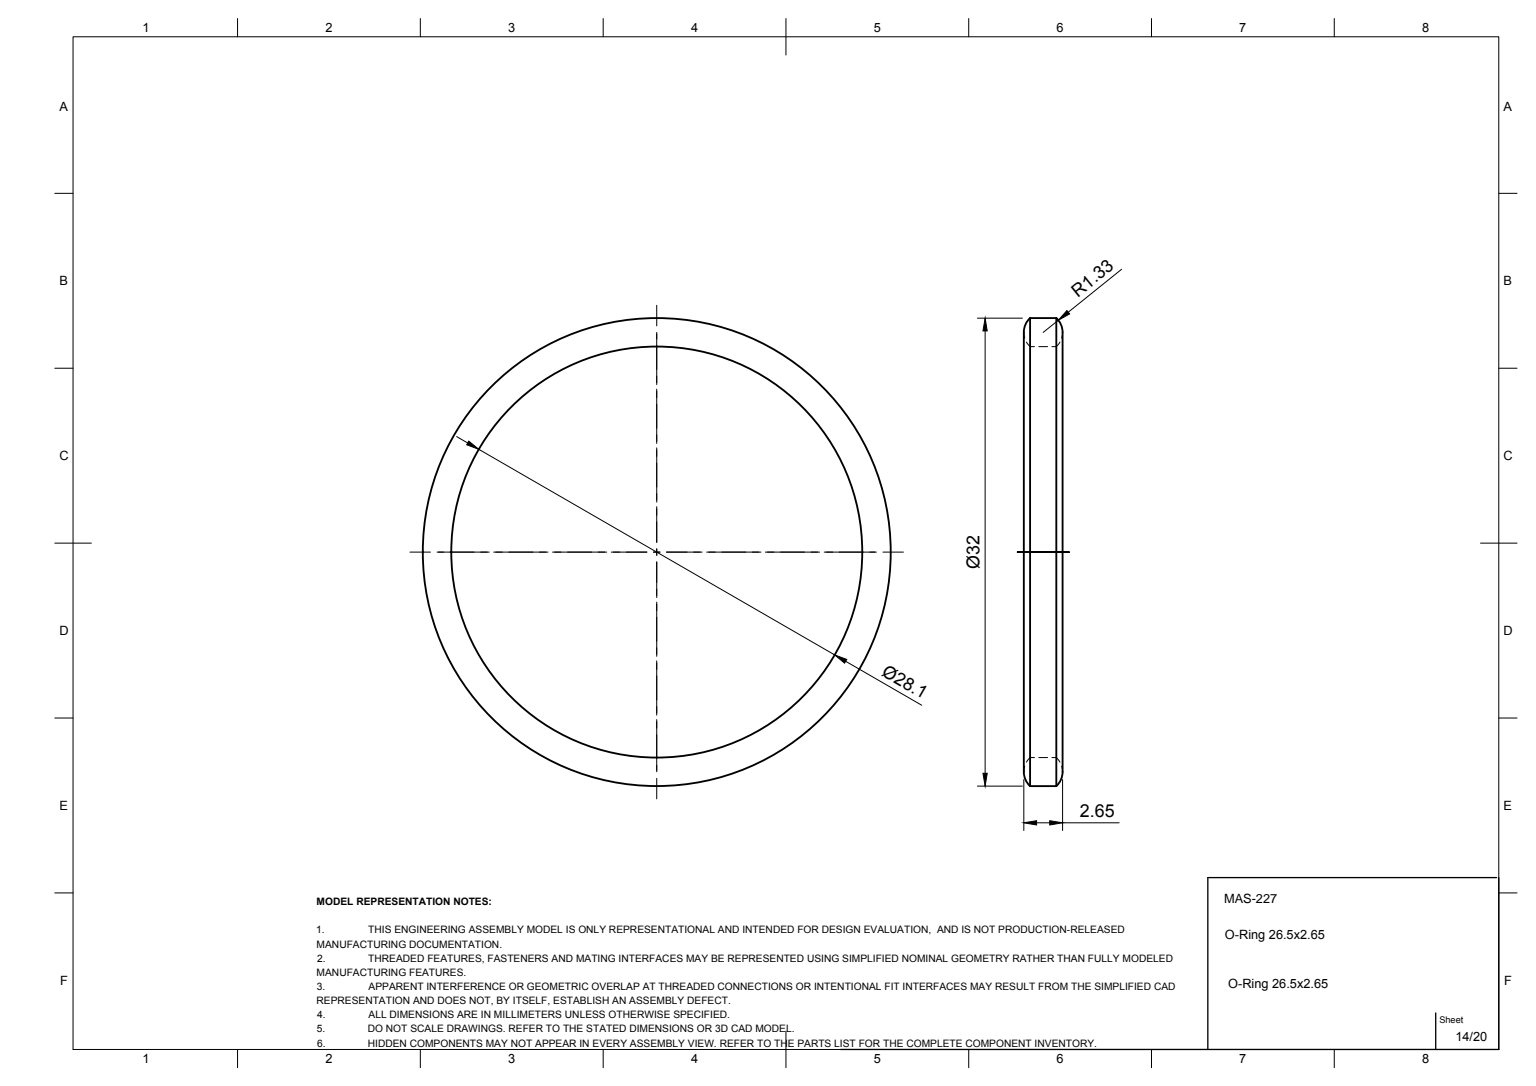
ISO-10303-21;
HEADER;
FILE_DESCRIPTION (('STEP AP214'),
    '1' );
FILE_NAME ( 'O-Ring 26.5x2.65.step', '2026-10-06T08:24:41', ( '' ), ( '' ), 'STEP AP214', 'Unspecified', '' );
FILE_SCHEMA (( 'AUTOMOTIVE_DESIGN' ));
ENDSEC;
DATA;
#16=VECTOR ( 'NONE', #25665, 39.37007874015748143 ) ;
#18=FACE_OUTER_BOUND ( 'NONE', #11254, .T. ) ;
#51=VERTEX_POINT ( 'NONE', #494 ) ;
#141=TOROIDAL_SURFACE ( 'NONE', #14548, 0.5915354330708662012, 0.05216535433070866590 ) ;
#282=DIRECTION ( 'NONE',  ( -5.737213000000000442E-16, 1.000000000000000000, -1.224646799147353207E-16 ) ) ;
#369=CARTESIAN_POINT ( 'NONE',  ( -0.03532354024591771724, -0.6299212598425195653, 0.6299212598425196763 ) ) ;
#494=CARTESIAN_POINT ( 'NONE',  ( -0.03532354024591775193, -0.07677165354330710290, 0.000000000000000000 ) ) ;
#622=CLOSED_SHELL ( 'NONE', ( #8560, #18644, #16249, #1256, #26576, #22771, #9012, #3173 ) ) ;
#701=EDGE_CURVE ( 'NONE', #51, #18891, #12838, .T. ) ;
#703=CARTESIAN_POINT ( 'NONE',  ( 0.03532354024591842501, -0.6299212598425196763, 0.000000000000000000 ) ) ;
#723=EDGE_CURVE ( 'NONE', #11887, #24760, #20053, .T. ) ;
#745=LINE ( 'NONE', #11474, #16 ) ;
#917=CARTESIAN_POINT ( 'NONE',  ( 3.387491338582676985E-16, -0.6299212598425196763, 0.000000000000000000 ) ) ;
#1221=PRODUCT_DEFINITION_SHAPE ( 'NONE', 'NONE',  #2566 ) ;
#1256=ADVANCED_FACE ( 'NONE', ( #5909 ), #16077, .T. ) ;
#1277=DIRECTION ( 'NONE',  ( 1.000000000000000000, 0.000000000000000000, 0.000000000000000000 ) ) ;
#1308=ORIENTED_EDGE ( 'NONE', *, *, #23601, .T. ) ;
#1320=EDGE_CURVE ( 'NONE', #51, #1745, #8572, .T. ) ;
#1375=DIRECTION ( 'NONE',  ( 5.737213000000000442E-16, -1.000000000000000000, 0.000000000000000000 ) ) ;
#1377=EDGE_CURVE ( 'NONE', #25529, #10943, #6997, .T. ) ;
#1378=DIRECTION ( 'NONE',  ( 1.000000000000000000, 0.000000000000000000, 0.000000000000000000 ) ) ;
#1561=CARTESIAN_POINT ( 'NONE',  ( 0.03532354024591839031, -0.6299212598425196763, -0.5531496062992127261 ) ) ;
#1621=ORIENTED_EDGE ( 'NONE', *, *, #19395, .F. ) ;
#1686=DIRECTION ( 'NONE',  ( -5.737213000000000442E-16, 1.000000000000000000, -1.224646799147353207E-16 ) ) ;
#1727=LINE ( 'NONE', #7814, #20994 ) ;
#1729=ORIENTED_EDGE ( 'NONE', *, *, #3922, .F. ) ;
#1745=VERTEX_POINT ( 'NONE', #5410 ) ;
#1841=CIRCLE ( 'NONE', #24842, 0.5531496062992126150 ) ;
#1899=SURFACE_SIDE_STYLE ('',( #20830 ) ) ;
#1912=DIRECTION ( 'NONE',  ( 1.000000000000000000, 0.000000000000000000, 0.000000000000000000 ) ) ;
#2140=DIRECTION ( 'NONE',  ( 0.000000000000000000, 1.000000000000000000, 0.000000000000000000 ) ) ;
#2162=AXIS2_PLACEMENT_3D ( 'NONE', #917, #9504, #7127 ) ;
#2367=CIRCLE ( 'NONE', #19974, 0.6299212598425196763 ) ;
#2507=CARTESIAN_POINT ( 'NONE',  ( 0.03532354024591842501, 0.000000000000000000, 0.000000000000000000 ) ) ;
#2559=EDGE_CURVE ( 'NONE', #27334, #51, #15612, .T. ) ;
#2561=CARTESIAN_POINT ( 'NONE',  ( 3.387491338582676985E-16, -0.6299212598425196763, 0.000000000000000000 ) ) ;
#2566=PRODUCT_DEFINITION ( 'UNKNOWN', '', #22916, #5726 ) ;
#2676=DIRECTION ( 'NONE',  ( 0.000000000000000000, 1.000000000000000000, 0.000000000000000000 ) ) ;
#3100=CYLINDRICAL_SURFACE ( 'NONE', #26407, 0.6299212598425196763 ) ;
#3173=ADVANCED_FACE ( 'NONE', ( #17968 ), #22023, .T. ) ;
#3194=DIRECTION ( 'NONE',  ( 0.000000000000000000, 1.000000000000000000, 0.000000000000000000 ) ) ;
#3206=DIRECTION ( 'NONE',  ( 0.000000000000000000, 1.000000000000000000, 0.000000000000000000 ) ) ;
#3358=DIRECTION ( 'NONE',  ( 0.000000000000000000, 1.000000000000000000, 0.000000000000000000 ) ) ;
#3457=DIRECTION ( 'NONE',  ( 5.737213000000000442E-16, -1.000000000000000000, 0.000000000000000000 ) ) ;
#3491=CYLINDRICAL_SURFACE ( 'NONE', #18443, 0.5531496062992126150 ) ;
#3649=APPLICATION_CONTEXT ( 'automotive_design' ) ;
#3665=DIRECTION ( 'NONE',  ( 0.000000000000000000, 0.000000000000000000, 1.000000000000000000 ) ) ;
#3722=CIRCLE ( 'NONE', #22210, 0.6299212598425196763 ) ;
#3837=CIRCLE ( 'NONE', #25481, 0.6299212598425196763 ) ;
#3861=EDGE_CURVE ( 'NONE', #26623, #1745, #13934, .T. ) ;
#3922=EDGE_CURVE ( 'NONE', #11887, #24839, #745, .T. ) ;
#3923=CIRCLE ( 'NONE', #15647, 0.5531496062992126150 ) ;
#3950=DIRECTION ( 'NONE',  ( 1.000000000000000000, 0.000000000000000000, 0.000000000000000000 ) ) ;
#3983=ORIENTED_EDGE ( 'NONE', *, *, #3922, .T. ) ;
#4113=ORIENTED_EDGE ( 'NONE', *, *, #7145, .F. ) ;
#4133=ORIENTED_EDGE ( 'NONE', *, *, #2559, .T. ) ;
#4199=CARTESIAN_POINT ( 'NONE',  ( 0.03532354024591839031, -0.6299212598425196763, 0.000000000000000000 ) ) ;
#4249=CIRCLE ( 'NONE', #25904, 0.05216535433070866590 ) ;
#4542=DIRECTION ( 'NONE',  ( 1.000000000000000000, 0.000000000000000000, 0.000000000000000000 ) ) ;
#4793=DIRECTION ( 'NONE',  ( 1.000000000000000000, 0.000000000000000000, 0.000000000000000000 ) ) ;
#4849=ORIENTED_EDGE ( 'NONE', *, *, #1377, .T. ) ;
#5188=ORIENTED_EDGE ( 'NONE', *, *, #10508, .T. ) ;
#5229=CARTESIAN_POINT ( 'NONE',  ( 0.000000000000000000, 0.000000000000000000, 0.000000000000000000 ) ) ;
#5323=CARTESIAN_POINT ( 'NONE',  ( 0.03532354024591842501, -0.6299212598425196763, 0.000000000000000000 ) ) ;
#5348=ORIENTED_EDGE ( 'NONE', *, *, #9549, .T. ) ;
#5410=CARTESIAN_POINT ( 'NONE',  ( 0.03532354024591839031, -0.07677165354330710290, 0.000000000000000000 ) ) ;
#5496=ORIENTED_EDGE ( 'NONE', *, *, #25810, .T. ) ;
#5510=PRODUCT ( 'O-Ring 26.5x2.65', 'O-Ring 26.5x2.65', '', ( #21672 ) ) ;
#5527=EDGE_CURVE ( 'NONE', #24760, #25529, #17543, .T. ) ;
#5576=AXIS2_PLACEMENT_3D ( 'NONE', #16947, #3950, #3358 ) ;
#5726=PRODUCT_DEFINITION_CONTEXT ( 'detailed design', #25319, 'design' ) ;
#5782=CARTESIAN_POINT ( 'NONE',  ( 3.168943700787402105E-16, -0.6299212598425196763, 0.000000000000000000 ) ) ;
#5828=CIRCLE ( 'NONE', #11673, 0.5531496062992126150 ) ;
#5871=ORIENTED_EDGE ( 'NONE', *, *, #7145, .T. ) ;
#5874=PRESENTATION_STYLE_ASSIGNMENT (( #23395 ) ) ;
#5909=FACE_OUTER_BOUND ( 'NONE', #24647, .T. ) ;
#5934=CARTESIAN_POINT ( 'NONE',  ( 0.03532354024591842501, -1.259842519685039353, 7.714310545810098438E-17 ) ) ;
#5938=LINE ( 'NONE', #7912, #15070 ) ;
#6195=DIMENSIONAL_EXPONENTS ( 1.000000000000000000, 0.000000000000000000, 0.000000000000000000, 0.000000000000000000, 0.000000000000000000, 0.000000000000000000, 0.000000000000000000 ) ;
#6290=( LENGTH_UNIT ( ) NAMED_UNIT ( * ) SI_UNIT ( $, .METRE. ) ) ;
#6293=ORIENTED_EDGE ( 'NONE', *, *, #24317, .F. ) ;
#6388=STYLED_ITEM ( 'NONE', ( #5874 ), #12535 ) ;
#6407=ORIENTED_EDGE ( 'NONE', *, *, #24317, .T. ) ;
#6613=ORIENTED_EDGE ( 'NONE', *, *, #9048, .F. ) ;
#6845=MECHANICAL_DESIGN_GEOMETRIC_PRESENTATION_REPRESENTATION('',(#6388),#8635);
#6878=ORIENTED_EDGE ( 'NONE', *, *, #1320, .T. ) ;
#6892=ORIENTED_EDGE ( 'NONE', *, *, #24202, .T. ) ;
#6938=CARTESIAN_POINT ( 'NONE',  ( 0.03532354024591839031, -1.183070866141732402, 6.774128948039492984E-17 ) ) ;
#6978=AXIS2_PLACEMENT_3D ( 'NONE', #20907, #22894, #25283 ) ;
#6997=CIRCLE ( 'NONE', #24127, 0.6299212598425196763 ) ;
#7054=CARTESIAN_POINT ( 'NONE',  ( -0.03532354024591775193, -1.183070866141732402, 6.774128948039492984E-17 ) ) ;
#7127=DIRECTION ( 'NONE',  ( 0.000000000000000000, 0.000000000000000000, -1.000000000000000000 ) ) ;
#7145=EDGE_CURVE ( 'NONE', #18891, #19141, #26171, .T. ) ;
#7197=FACE_OUTER_BOUND ( 'NONE', #21819, .T. ) ;
#7289=DIRECTION ( 'NONE',  ( 0.000000000000000000, 1.000000000000000000, 0.000000000000000000 ) ) ;
#7307=AXIS2_PLACEMENT_3D ( 'NONE', #9577, #20051, #20188 ) ;
#7358=CARTESIAN_POINT ( 'NONE',  ( 3.606039370078740678E-16, -0.6299212598425196763, 0.000000000000000000 ) ) ;
#7437=DIRECTION ( 'NONE',  ( 1.000000000000000000, 0.000000000000000000, 0.000000000000000000 ) ) ;
#7561=ORIENTED_EDGE ( 'NONE', *, *, #20852, .T. ) ;
#7745=DIRECTION ( 'NONE',  ( 0.000000000000000000, 1.000000000000000000, 0.000000000000000000 ) ) ;
#7814=CARTESIAN_POINT ( 'NONE',  ( 3.606039370078740678E-16, 0.000000000000000000, 0.000000000000000000 ) ) ;
#7894=DIRECTION ( 'NONE',  ( 1.000000000000000000, 0.000000000000000000, 0.000000000000000000 ) ) ;
#7912=CARTESIAN_POINT ( 'NONE',  ( 3.168943700787402105E-16, -1.183070866141732402, 6.774128948039492984E-17 ) ) ;
#7923=DIRECTION ( 'NONE',  ( 1.000000000000000000, 0.000000000000000000, 0.000000000000000000 ) ) ;
#8115=CARTESIAN_POINT ( 'NONE',  ( -0.03532354024591771724, -0.6299212598425196763, 0.000000000000000000 ) ) ;
#8193=DIRECTION ( 'NONE',  ( -1.000000000000000000, 0.000000000000000000, 0.000000000000000000 ) ) ;
#8226=CARTESIAN_POINT ( 'NONE',  ( -0.03532354024591775193, -0.6299212598425196763, 0.000000000000000000 ) ) ;
#8367=AXIS2_PLACEMENT_3D ( 'NONE', #19784, #4793, #2676 ) ;
#8370=DIRECTION ( 'NONE',  ( 0.000000000000000000, 1.000000000000000000, 0.000000000000000000 ) ) ;
#8452=ORIENTED_EDGE ( 'NONE', *, *, #15845, .T. ) ;
#8560=ADVANCED_FACE ( 'NONE', ( #10919 ), #141, .T. ) ;
#8572=LINE ( 'NONE', #21570, #16465 ) ;
#8584=( LENGTH_UNIT ( ) NAMED_UNIT ( * ) SI_UNIT ( $, .METRE. ) ) ;
#8595=CARTESIAN_POINT ( 'NONE',  ( -0.03532354024591775193, -0.6299212598425196763, 0.000000000000000000 ) ) ;
#8635=( GEOMETRIC_REPRESENTATION_CONTEXT ( 3 ) GLOBAL_UNCERTAINTY_ASSIGNED_CONTEXT ( ( #20622 ) ) GLOBAL_UNIT_ASSIGNED_CONTEXT ( ( #10223, #14502, #18839 ) ) REPRESENTATION_CONTEXT ( 'NONE', 'WORKASPACE' ) ) ;
#8706=ORIENTED_EDGE ( 'NONE', *, *, #3861, .T. ) ;
#8817=ORIENTED_EDGE ( 'NONE', *, *, #3861, .F. ) ;
#8923=DIRECTION ( 'NONE',  ( 1.000000000000000000, 5.737213000000000442E-16, 0.000000000000000000 ) ) ;
#8965=AXIS2_PLACEMENT_3D ( 'NONE', #10400, #14533, #19018 ) ;
#9012=ADVANCED_FACE ( 'NONE', ( #7197 ), #18185, .F. ) ;
#9048=EDGE_CURVE ( 'NONE', #19937, #24839, #3722, .T. ) ;
#9159=TOROIDAL_SURFACE ( 'NONE', #15501, 0.5915354330708662012, 0.05216535433070866590 ) ;
#9460=TOROIDAL_SURFACE ( 'NONE', #18012, 0.5915354330708662012, 0.05216535433070866590 ) ;
#9504=DIRECTION ( 'NONE',  ( 1.000000000000000000, 5.737213000000000442E-16, 0.000000000000000000 ) ) ;
#9549=EDGE_CURVE ( 'NONE', #10943, #11887, #2367, .T. ) ;
#9577=CARTESIAN_POINT ( 'NONE',  ( 3.168943700787402105E-16, -0.6299212598425196763, 0.000000000000000000 ) ) ;
#9708=CARTESIAN_POINT ( 'NONE',  ( -0.03532354024591771724, -0.6299212598425196763, 0.000000000000000000 ) ) ;
#10152=CARTESIAN_POINT ( 'NONE',  ( 3.387491338582676492E-16, -0.6299212598425195653, 0.5915354330708662012 ) ) ;
#10223=( CONVERSION_BASED_UNIT ( 'INCH', #18990 ) LENGTH_UNIT ( ) NAMED_UNIT ( #6195 ) ) ;
#10261=DIRECTION ( 'NONE',  ( 1.000000000000000000, 0.000000000000000000, 0.000000000000000000 ) ) ;
#10400=CARTESIAN_POINT ( 'NONE',  ( 0.03532354024591839031, -0.6299212598425196763, 0.000000000000000000 ) ) ;
#10445=COLOUR_RGB ( '', 0.31764706, 0.68627451, 0.89019608) ;
#10475=AXIS2_PLACEMENT_3D ( 'NONE', #19178, #282, #16785 ) ;
#10508=EDGE_CURVE ( 'NONE', #18891, #10943, #22660, .T. ) ;
#10552=( NAMED_UNIT ( * ) PLANE_ANGLE_UNIT ( ) SI_UNIT ( $, .RADIAN. ) ) ;
#10610=DIRECTION ( 'NONE',  ( 1.000000000000000000, 0.000000000000000000, 0.000000000000000000 ) ) ;
#10700=( NAMED_UNIT ( * ) SI_UNIT ( $, .STERADIAN. ) SOLID_ANGLE_UNIT ( ) ) ;
#10913=ORIENTED_EDGE ( 'NONE', *, *, #701, .T. ) ;
#10919=FACE_OUTER_BOUND ( 'NONE', #21859, .T. ) ;
#10943=VERTEX_POINT ( 'NONE', #369 ) ;
#11074=CIRCLE ( 'NONE', #8367, 0.6299212598425196763 ) ;
#11125=DIRECTION ( 'NONE',  ( 0.000000000000000000, 1.000000000000000000, 0.000000000000000000 ) ) ;
#11254=EDGE_LOOP ( 'NONE', ( #27328, #5871, #12556, #15233, #16781, #13315 ) ) ;
#11343=ORIENTED_EDGE ( 'NONE', *, *, #1377, .F. ) ;
#11417=ORIENTED_EDGE ( 'NONE', *, *, #25810, .F. ) ;
#11474=CARTESIAN_POINT ( 'NONE',  ( 3.606039370078740678E-16, -1.259842519685039353, 7.714310545810098438E-17 ) ) ;
#11588=AXIS2_PLACEMENT_3D ( 'NONE', #5229, #3665, #7923 ) ;
#11673=AXIS2_PLACEMENT_3D ( 'NONE', #27494, #1912, #14660 ) ;
#11887=VERTEX_POINT ( 'NONE', #20844 ) ;
#12159=EDGE_CURVE ( 'NONE', #22507, #26151, #1841, .T. ) ;
#12245=ORIENTED_EDGE ( 'NONE', *, *, #701, .F. ) ;
#12535=MANIFOLD_SOLID_BREP ( 'O-Ring 26.5x2.65', #622 ) ;
#12556=ORIENTED_EDGE ( 'NONE', *, *, #18908, .T. ) ;
#12838=CIRCLE ( 'NONE', #6978, 0.5531496062992126150 ) ;
#13036=DIRECTION ( 'NONE',  ( 1.000000000000000000, 5.737213000000000442E-16, 0.000000000000000000 ) ) ;
#13038=ORIENTED_EDGE ( 'NONE', *, *, #20852, .F. ) ;
#13084=ORIENTED_EDGE ( 'NONE', *, *, #25064, .T. ) ;
#13315=ORIENTED_EDGE ( 'NONE', *, *, #9549, .F. ) ;
#13403=DIMENSIONAL_EXPONENTS ( 1.000000000000000000, 0.000000000000000000, 0.000000000000000000, 0.000000000000000000, 0.000000000000000000, 0.000000000000000000, 0.000000000000000000 ) ;
#13446=EDGE_CURVE ( 'NONE', #19463, #18018, #19077, .T. ) ;
#13454=AXIS2_PLACEMENT_3D ( 'NONE', #9708, #20867, #3194 ) ;
#13637=ORIENTED_EDGE ( 'NONE', *, *, #12159, .F. ) ;
#13748=ORIENTED_EDGE ( 'NONE', *, *, #2559, .F. ) ;
#13856=DIRECTION ( 'NONE',  ( 0.000000000000000000, 1.000000000000000000, 0.000000000000000000 ) ) ;
#13932=CARTESIAN_POINT ( 'NONE',  ( -0.03532354024591775193, -0.6299212598425196763, 0.000000000000000000 ) ) ;
#13934=CIRCLE ( 'NONE', #8965, 0.5531496062992126150 ) ;
#14012=EDGE_CURVE ( 'NONE', #19141, #26151, #5938, .T. ) ;
#14091=DIRECTION ( 'NONE',  ( 1.000000000000000000, 0.000000000000000000, 0.000000000000000000 ) ) ;
#14222=AXIS2_PLACEMENT_3D ( 'NONE', #16221, #1378, #7745 ) ;
#14424=DIRECTION ( 'NONE',  ( 1.000000000000000000, 0.000000000000000000, 0.000000000000000000 ) ) ;
#14502=( NAMED_UNIT ( * ) PLANE_ANGLE_UNIT ( ) SI_UNIT ( $, .RADIAN. ) ) ;
#14533=DIRECTION ( 'NONE',  ( 1.000000000000000000, 0.000000000000000000, 0.000000000000000000 ) ) ;
#14548=AXIS2_PLACEMENT_3D ( 'NONE', #2561, #13036, #19808 ) ;
#14660=DIRECTION ( 'NONE',  ( 0.000000000000000000, 1.000000000000000000, 0.000000000000000000 ) ) ;
#14685=DIRECTION ( 'NONE',  ( 0.000000000000000000, 1.000000000000000000, 0.000000000000000000 ) ) ;
#14716=EDGE_LOOP ( 'NONE', ( #24966, #25552, #7561, #8706, #23121, #13748 ) ) ;
#14734=AXIS2_PLACEMENT_3D ( 'NONE', #8226, #4542, #8370 ) ;
#14830=DIRECTION ( 'NONE',  ( 1.000000000000000000, 5.737213000000000442E-16, 0.000000000000000000 ) ) ;
#15070=VECTOR ( 'NONE', #14424, 39.37007874015748143 ) ;
#15138=ORIENTED_EDGE ( 'NONE', *, *, #13446, .F. ) ;
#15233=ORIENTED_EDGE ( 'NONE', *, *, #19395, .T. ) ;
#15501=AXIS2_PLACEMENT_3D ( 'NONE', #23441, #14830, #25820 ) ;
#15612=CIRCLE ( 'NONE', #14734, 0.5531496062992126150 ) ;
#15647=AXIS2_PLACEMENT_3D ( 'NONE', #13932, #25725, #7289 ) ;
#15747=CARTESIAN_POINT ( 'NONE',  ( -0.03532354024591775193, -0.6299212598425196763, -0.5531496062992126150 ) ) ;
#15817=DIRECTION ( 'NONE',  ( 1.000000000000000000, 0.000000000000000000, 0.000000000000000000 ) ) ;
#15845=EDGE_CURVE ( 'NONE', #25529, #18018, #1727, .T. ) ;
#15977=DIRECTION ( 'NONE',  ( 1.000000000000000000, 0.000000000000000000, 0.000000000000000000 ) ) ;
#16077=CYLINDRICAL_SURFACE ( 'NONE', #14222, 0.6299212598425196763 ) ;
#16221=CARTESIAN_POINT ( 'NONE',  ( 3.606039370078740678E-16, -0.6299212598425196763, 0.000000000000000000 ) ) ;
#16249=ADVANCED_FACE ( 'NONE', ( #21656 ), #9460, .T. ) ;
#16465=VECTOR ( 'NONE', #10261, 39.37007874015748143 ) ;
#16570=( GEOMETRIC_REPRESENTATION_CONTEXT ( 3 ) GLOBAL_UNCERTAINTY_ASSIGNED_CONTEXT ( ( #23243 ) ) GLOBAL_UNIT_ASSIGNED_CONTEXT ( ( #25683, #10552, #10700 ) ) REPRESENTATION_CONTEXT ( 'NONE', 'WORKASPACE' ) ) ;
#16606=DIRECTION ( 'NONE',  ( 1.000000000000000000, 0.000000000000000000, 0.000000000000000000 ) ) ;
#16655=ORIENTED_EDGE ( 'NONE', *, *, #9048, .T. ) ;
#16781=ORIENTED_EDGE ( 'NONE', *, *, #723, .F. ) ;
#16785=DIRECTION ( 'NONE',  ( -1.000000000000000000, 0.000000000000000000, 0.000000000000000000 ) ) ;
#16820=ORIENTED_EDGE ( 'NONE', *, *, #14012, .F. ) ;
#16855=DIRECTION ( 'NONE',  ( 1.000000000000000000, 0.000000000000000000, 0.000000000000000000 ) ) ;
#16933=ORIENTED_EDGE ( 'NONE', *, *, #723, .T. ) ;
#16947=CARTESIAN_POINT ( 'NONE',  ( 0.03532354024591839031, -0.6299212598425196763, 0.000000000000000000 ) ) ;
#17115=EDGE_LOOP ( 'NONE', ( #4133, #10913, #5188, #11343, #21481, #1621 ) ) ;
#17259=CARTESIAN_POINT ( 'NONE',  ( 0.03532354024591842501, -0.6299212598425196763, 0.000000000000000000 ) ) ;
#17353=DIRECTION ( 'NONE',  ( 1.000000000000000000, 0.000000000000000000, 0.000000000000000000 ) ) ;
#17473=ORIENTED_EDGE ( 'NONE', *, *, #12159, .T. ) ;
#17543=CIRCLE ( 'NONE', #13454, 0.6299212598425196763 ) ;
#17968=FACE_OUTER_BOUND ( 'NONE', #26843, .T. ) ;
#17990=CARTESIAN_POINT ( 'NONE',  ( 0.03532354024591842501, -0.6299212598425196763, -0.6299212598425196763 ) ) ;
#18012=AXIS2_PLACEMENT_3D ( 'NONE', #19676, #8923, #26164 ) ;
#18018=VERTEX_POINT ( 'NONE', #2507 ) ;
#18054=FACE_OUTER_BOUND ( 'NONE', #27815, .T. ) ;
#18185=CYLINDRICAL_SURFACE ( 'NONE', #7307, 0.5531496062992126150 ) ;
#18443=AXIS2_PLACEMENT_3D ( 'NONE', #5782, #7894, #3206 ) ;
#18644=ADVANCED_FACE ( 'NONE', ( #26812 ), #3491, .F. ) ;
#18649=CARTESIAN_POINT ( 'NONE',  ( -0.03532354024591771724, 0.000000000000000000, 0.000000000000000000 ) ) ;
#18757=CIRCLE ( 'NONE', #21475, 0.05216535433070866590 ) ;
#18767=ADVANCED_BREP_SHAPE_REPRESENTATION ( 'O-Ring 26.5x2.65', ( #12535, #11588 ), #16570 ) ;
#18839=( NAMED_UNIT ( * ) SI_UNIT ( $, .STERADIAN. ) SOLID_ANGLE_UNIT ( ) ) ;
#18891=VERTEX_POINT ( 'NONE', #26884 ) ;
#18896=ORIENTED_EDGE ( 'NONE', *, *, #5527, .T. ) ;
#18905=ORIENTED_EDGE ( 'NONE', *, *, #13446, .T. ) ;
#18908=EDGE_CURVE ( 'NONE', #19141, #27334, #3923, .T. ) ;
#18960=CARTESIAN_POINT ( 'NONE',  ( 0.03532354024591842501, -0.6299212598425195653, 0.6299212598425196763 ) ) ;
#18990=LENGTH_MEASURE_WITH_UNIT ( LENGTH_MEASURE( 0.02539999999999999897 ), #6290 ) ;
#19018=DIRECTION ( 'NONE',  ( 0.000000000000000000, 1.000000000000000000, 0.000000000000000000 ) ) ;
#19077=CIRCLE ( 'NONE', #22216, 0.6299212598425196763 ) ;
#19141=VERTEX_POINT ( 'NONE', #7054 ) ;
#19176=SHAPE_REPRESENTATION_RELATIONSHIP ( 'NONE' , 'NONE' ,  #27787, #18767 ) ;
#19178=CARTESIAN_POINT ( 'NONE',  ( 3.387491338582676492E-16, -0.6299212598425195653, 0.5915354330708662012 ) ) ;
#19395=EDGE_CURVE ( 'NONE', #27334, #24760, #18757, .T. ) ;
#19463=VERTEX_POINT ( 'NONE', #17990 ) ;
#19676=CARTESIAN_POINT ( 'NONE',  ( 3.387491338582676985E-16, -0.6299212598425196763, 0.000000000000000000 ) ) ;
#19784=CARTESIAN_POINT ( 'NONE',  ( 0.03532354024591842501, -0.6299212598425196763, 0.000000000000000000 ) ) ;
#19808=DIRECTION ( 'NONE',  ( 0.000000000000000000, 0.000000000000000000, -1.000000000000000000 ) ) ;
#19937=VERTEX_POINT ( 'NONE', #18960 ) ;
#19974=AXIS2_PLACEMENT_3D ( 'NONE', #8115, #20819, #23093 ) ;
#20051=DIRECTION ( 'NONE',  ( 1.000000000000000000, 0.000000000000000000, 0.000000000000000000 ) ) ;
#20053=CIRCLE ( 'NONE', #20968, 0.6299212598425196763 ) ;
#20188=DIRECTION ( 'NONE',  ( 0.000000000000000000, 1.000000000000000000, 0.000000000000000000 ) ) ;
#20622=UNCERTAINTY_MEASURE_WITH_UNIT (LENGTH_MEASURE( 1.000000000000000082E-05 ), #10223, 'distance_accuracy_value', 'NONE') ;
#20786=ORIENTED_EDGE ( 'NONE', *, *, #15845, .F. ) ;
#20819=DIRECTION ( 'NONE',  ( 1.000000000000000000, 0.000000000000000000, 0.000000000000000000 ) ) ;
#20830=SURFACE_STYLE_FILL_AREA ( #27763 ) ;
#20844=CARTESIAN_POINT ( 'NONE',  ( -0.03532354024591771724, -1.259842519685039353, 7.714310545810098438E-17 ) ) ;
#20852=EDGE_CURVE ( 'NONE', #26151, #26623, #5828, .T. ) ;
#20867=DIRECTION ( 'NONE',  ( 1.000000000000000000, 0.000000000000000000, 0.000000000000000000 ) ) ;
#20907=CARTESIAN_POINT ( 'NONE',  ( -0.03532354024591775193, -0.6299212598425196763, 0.000000000000000000 ) ) ;
#20968=AXIS2_PLACEMENT_3D ( 'NONE', #25140, #1277, #22604 ) ;
#20994=VECTOR ( 'NONE', #16855, 39.37007874015748143 ) ;
#21019=LENGTH_MEASURE_WITH_UNIT ( LENGTH_MEASURE( 0.02539999999999999897 ), #8584 ) ;
#21475=AXIS2_PLACEMENT_3D ( 'NONE', #24819, #1375, #14091 ) ;
#21481=ORIENTED_EDGE ( 'NONE', *, *, #5527, .F. ) ;
#21570=CARTESIAN_POINT ( 'NONE',  ( 3.168943700787402105E-16, -0.07677165354330710290, 0.000000000000000000 ) ) ;
#21656=FACE_OUTER_BOUND ( 'NONE', #17115, .T. ) ;
#21672=PRODUCT_CONTEXT ( 'NONE', #3649, 'mechanical' ) ;
#21819=EDGE_LOOP ( 'NONE', ( #16820, #4113, #12245, #6878, #1308, #17473 ) ) ;
#21830=CIRCLE ( 'NONE', #24529, 0.05216535433070866590 ) ;
#21859=EDGE_LOOP ( 'NONE', ( #13084, #6892, #27343, #8817, #6293, #18905 ) ) ;
#21889=CARTESIAN_POINT ( 'NONE',  ( 0.03532354024591839031, -0.6299212598425196763, 0.5531496062992127261 ) ) ;
#22023=TOROIDAL_SURFACE ( 'NONE', #2162, 0.5915354330708662012, 0.05216535433070866590 ) ;
#22210=AXIS2_PLACEMENT_3D ( 'NONE', #703, #15817, #26678 ) ;
#22216=AXIS2_PLACEMENT_3D ( 'NONE', #17259, #10610, #2140 ) ;
#22507=VERTEX_POINT ( 'NONE', #21889 ) ;
#22604=DIRECTION ( 'NONE',  ( 0.000000000000000000, 1.000000000000000000, 0.000000000000000000 ) ) ;
#22660=CIRCLE ( 'NONE', #10475, 0.05216535433070866590 ) ;
#22771=ADVANCED_FACE ( 'NONE', ( #18 ), #9159, .T. ) ;
#22894=DIRECTION ( 'NONE',  ( 1.000000000000000000, 0.000000000000000000, 0.000000000000000000 ) ) ;
#22916=PRODUCT_DEFINITION_FORMATION_WITH_SPECIFIED_SOURCE ( 'ANY', '', #5510, .NOT_KNOWN. ) ;
#23093=DIRECTION ( 'NONE',  ( 0.000000000000000000, 1.000000000000000000, 0.000000000000000000 ) ) ;
#23121=ORIENTED_EDGE ( 'NONE', *, *, #1320, .F. ) ;
#23243=UNCERTAINTY_MEASURE_WITH_UNIT (LENGTH_MEASURE( 1.000000000000000082E-05 ), #25683, 'distance_accuracy_value', 'NONE') ;
#23291=CARTESIAN_POINT ( 'NONE',  ( -0.03532354024591771724, -0.6299212598425196763, 0.000000000000000000 ) ) ;
#23292=DIRECTION ( 'NONE',  ( 1.000000000000000000, 0.000000000000000000, 0.000000000000000000 ) ) ;
#23395=SURFACE_STYLE_USAGE ( .BOTH. , #1899 ) ;
#23430=DIRECTION ( 'NONE',  ( 1.000000000000000000, 0.000000000000000000, 0.000000000000000000 ) ) ;
#23441=CARTESIAN_POINT ( 'NONE',  ( 3.387491338582676985E-16, -0.6299212598425196763, 0.000000000000000000 ) ) ;
#23601=EDGE_CURVE ( 'NONE', #1745, #22507, #23641, .T. ) ;
#23641=CIRCLE ( 'NONE', #5576, 0.5531496062992126150 ) ;
#23926=AXIS2_PLACEMENT_3D ( 'NONE', #8595, #17353, #11125 ) ;
#24127=AXIS2_PLACEMENT_3D ( 'NONE', #23291, #23430, #14685 ) ;
#24202=EDGE_CURVE ( 'NONE', #19937, #22507, #21830, .T. ) ;
#24317=EDGE_CURVE ( 'NONE', #19463, #26623, #4249, .T. ) ;
#24529=AXIS2_PLACEMENT_3D ( 'NONE', #10152, #1686, #8193 ) ;
#24647=EDGE_LOOP ( 'NONE', ( #4849, #5348, #3983, #6613, #25488, #20786 ) ) ;
#24760=VERTEX_POINT ( 'NONE', #27545 ) ;
#24807=DIRECTION ( 'NONE',  ( 0.000000000000000000, 1.000000000000000000, 0.000000000000000000 ) ) ;
#24819=CARTESIAN_POINT ( 'NONE',  ( 3.387491338582676985E-16, -0.6299212598425196763, -0.5915354330708662012 ) ) ;
#24839=VERTEX_POINT ( 'NONE', #5934 ) ;
#24842=AXIS2_PLACEMENT_3D ( 'NONE', #4199, #23292, #25109 ) ;
#24966=ORIENTED_EDGE ( 'NONE', *, *, #18908, .F. ) ;
#25064=EDGE_CURVE ( 'NONE', #18018, #19937, #3837, .T. ) ;
#25109=DIRECTION ( 'NONE',  ( 0.000000000000000000, 1.000000000000000000, 0.000000000000000000 ) ) ;
#25140=CARTESIAN_POINT ( 'NONE',  ( -0.03532354024591771724, -0.6299212598425196763, 0.000000000000000000 ) ) ;
#25208=FILL_AREA_STYLE_COLOUR ( '', #10445 ) ;
#25283=DIRECTION ( 'NONE',  ( 0.000000000000000000, 1.000000000000000000, 0.000000000000000000 ) ) ;
#25319=APPLICATION_CONTEXT ( 'automotive_design' ) ;
#25481=AXIS2_PLACEMENT_3D ( 'NONE', #5323, #7437, #24807 ) ;
#25488=ORIENTED_EDGE ( 'NONE', *, *, #25064, .F. ) ;
#25529=VERTEX_POINT ( 'NONE', #18649 ) ;
#25552=ORIENTED_EDGE ( 'NONE', *, *, #14012, .T. ) ;
#25665=DIRECTION ( 'NONE',  ( 1.000000000000000000, 0.000000000000000000, 0.000000000000000000 ) ) ;
#25683=( CONVERSION_BASED_UNIT ( 'INCH', #21019 ) LENGTH_UNIT ( ) NAMED_UNIT ( #13403 ) ) ;
#25725=DIRECTION ( 'NONE',  ( 1.000000000000000000, 0.000000000000000000, 0.000000000000000000 ) ) ;
#25810=EDGE_CURVE ( 'NONE', #24839, #19463, #11074, .T. ) ;
#25820=DIRECTION ( 'NONE',  ( 0.000000000000000000, 0.000000000000000000, -1.000000000000000000 ) ) ;
#25904=AXIS2_PLACEMENT_3D ( 'NONE', #26394, #3457, #16606 ) ;
#26151=VERTEX_POINT ( 'NONE', #6938 ) ;
#26164=DIRECTION ( 'NONE',  ( 0.000000000000000000, 0.000000000000000000, -1.000000000000000000 ) ) ;
#26171=CIRCLE ( 'NONE', #23926, 0.5531496062992126150 ) ;
#26394=CARTESIAN_POINT ( 'NONE',  ( 3.387491338582676985E-16, -0.6299212598425196763, -0.5915354330708662012 ) ) ;
#26407=AXIS2_PLACEMENT_3D ( 'NONE', #7358, #15977, #13856 ) ;
#26576=ADVANCED_FACE ( 'NONE', ( #18054 ), #3100, .T. ) ;
#26582=SHAPE_DEFINITION_REPRESENTATION ( #1221, #27787 ) ;
#26623=VERTEX_POINT ( 'NONE', #1561 ) ;
#26670=ORIENTED_EDGE ( 'NONE', *, *, #24202, .F. ) ;
#26678=DIRECTION ( 'NONE',  ( 0.000000000000000000, 1.000000000000000000, 0.000000000000000000 ) ) ;
#26812=FACE_OUTER_BOUND ( 'NONE', #14716, .T. ) ;
#26843=EDGE_LOOP ( 'NONE', ( #26670, #16655, #5496, #6407, #13038, #13637 ) ) ;
#26884=CARTESIAN_POINT ( 'NONE',  ( -0.03532354024591775193, -0.6299212598425196763, 0.5531496062992126150 ) ) ;
#27328=ORIENTED_EDGE ( 'NONE', *, *, #10508, .F. ) ;
#27334=VERTEX_POINT ( 'NONE', #15747 ) ;
#27343=ORIENTED_EDGE ( 'NONE', *, *, #23601, .F. ) ;
#27494=CARTESIAN_POINT ( 'NONE',  ( 0.03532354024591839031, -0.6299212598425196763, 0.000000000000000000 ) ) ;
#27545=CARTESIAN_POINT ( 'NONE',  ( -0.03532354024591771724, -0.6299212598425196763, -0.6299212598425196763 ) ) ;
#27763=FILL_AREA_STYLE ('',( #25208 ) ) ;
#27787=SHAPE_REPRESENTATION ( 'O-Ring 26.5x2.65', ( #11588 ), #16570 ) ;
#27815=EDGE_LOOP ( 'NONE', ( #1729, #16933, #18896, #8452, #15138, #11417 ) ) ;
ENDSEC;
END-ISO-10303-21;
